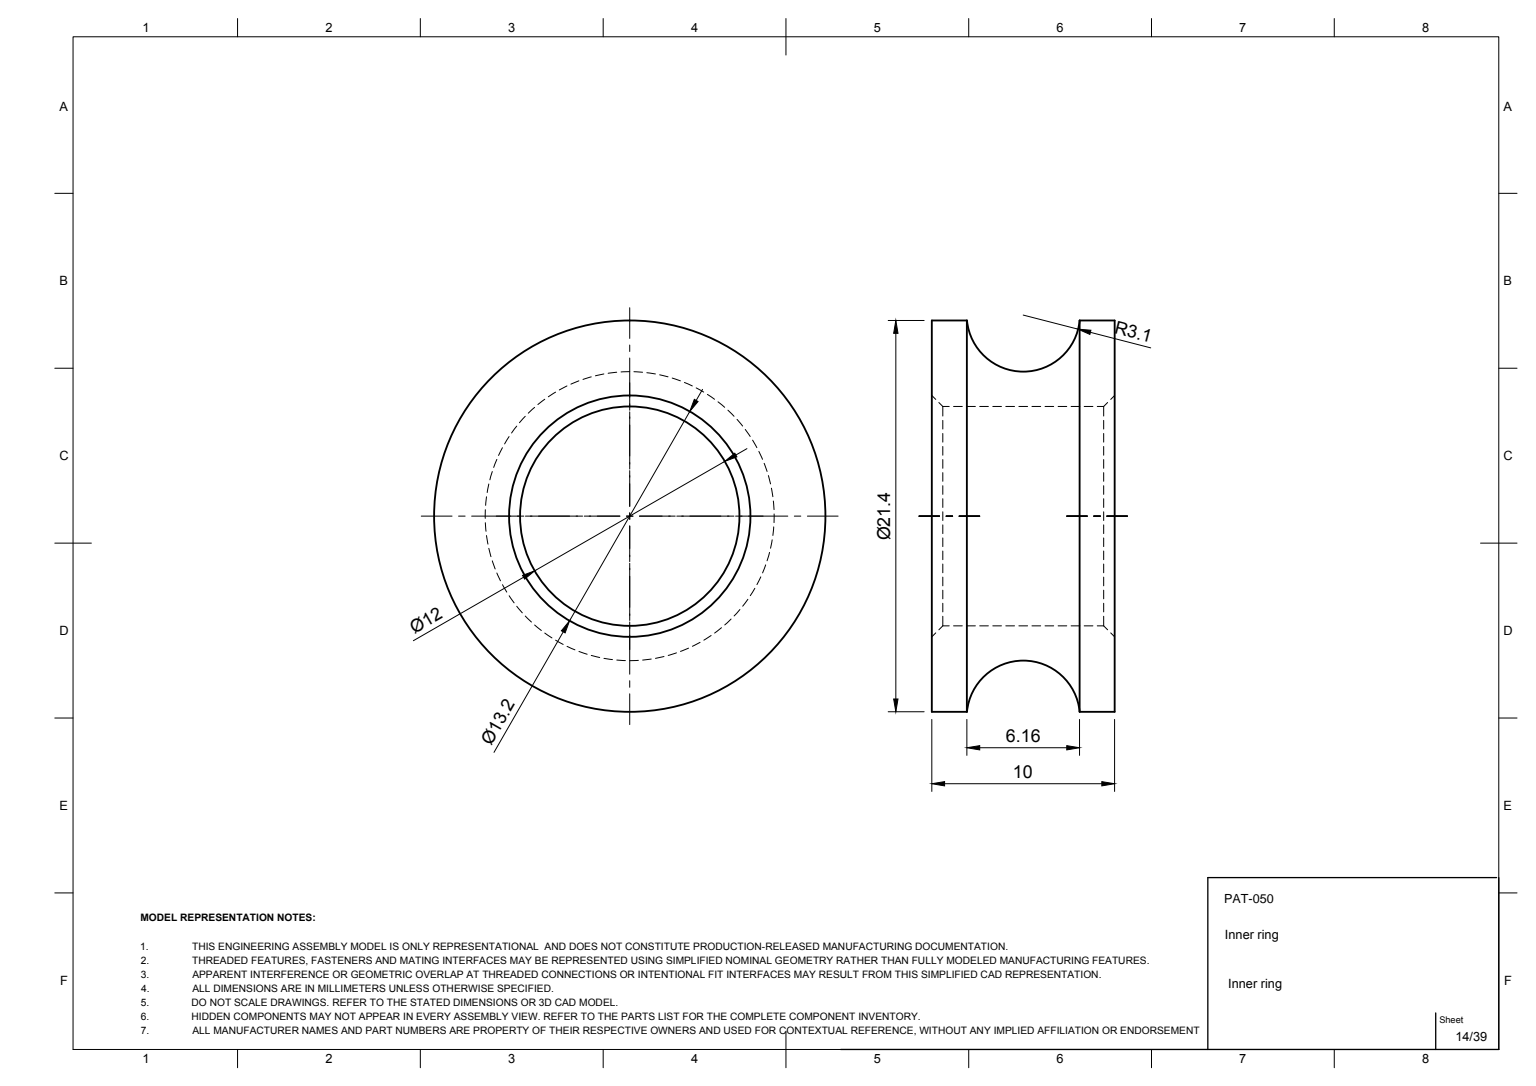
ISO-10303-21;
HEADER;
/* Generated by software containing ST-Developer
 * from STEP Tools, Inc. (www.steptools.com) 
 */

FILE_DESCRIPTION(
/* description */ ('Hand wheel with handle and shaft collar'),
/* implementation_level */ '2;1');

FILE_NAME(
/* name */ 'Inner ring.step',
/* time_stamp */ '2026-10-28T03:23:19-07:00',
/* author */ (''),
/* organization */ (''),
/* preprocessor_version */ 'ST-DEVELOPER v20.2',
/* originating_system */ 'Autodesk Translation Framework v15.17.0.0',
/* authorisation */ '');

FILE_SCHEMA (('AUTOMOTIVE_DESIGN { 1 0 10303 214 3 1 1 }'));
ENDSEC;

DATA;
#10=MECHANICAL_DESIGN_GEOMETRIC_PRESENTATION_REPRESENTATION('',(#404),#10510);
#297=TOROIDAL_SURFACE('',#5864,1.1,0.309556);
#304=CONICAL_SURFACE('',#5875,0.63,0.785398163397448);
#305=CONICAL_SURFACE('',#5882,0.63,0.785398163397448);
#340=SHAPE_REPRESENTATION_RELATIONSHIP('SRR','None',#10657,#372);
#372=ADVANCED_BREP_SHAPE_REPRESENTATION('',(#450),#10484);
#404=STYLED_ITEM('',(#10908),#450);
#450=MANIFOLD_SOLID_BREP('Body1',#5304);
#539=FACE_BOUND('',#1225,.T.);
#540=FACE_BOUND('',#1228,.T.);
#647=PLANE('',#5877);
#648=PLANE('',#5880);
#848=FACE_OUTER_BOUND('',#1220,.T.);
#849=FACE_OUTER_BOUND('',#1221,.T.);
#850=FACE_OUTER_BOUND('',#1222,.T.);
#851=FACE_OUTER_BOUND('',#1223,.T.);
#852=FACE_OUTER_BOUND('',#1224,.T.);
#853=FACE_OUTER_BOUND('',#1226,.T.);
#854=FACE_OUTER_BOUND('',#1227,.T.);
#855=FACE_OUTER_BOUND('',#1229,.T.);
#1220=EDGE_LOOP('',(#3923,#3924,#3925,#3926,#3927,#3928));
#1221=EDGE_LOOP('',(#3929,#3930,#3931,#3932,#3933));
#1222=EDGE_LOOP('',(#3934,#3935,#3936,#3937));
#1223=EDGE_LOOP('',(#3938,#3939,#3940,#3941));
#1224=EDGE_LOOP('',(#3942));
#1225=EDGE_LOOP('',(#3943));
#1226=EDGE_LOOP('',(#3944,#3945,#3946,#3947,#3948));
#1227=EDGE_LOOP('',(#3949));
#1228=EDGE_LOOP('',(#3950));
#1229=EDGE_LOOP('',(#3951,#3952,#3953,#3954));
#1627=LINE('',#8587,#1937);
#1628=LINE('',#8593,#1938);
#1629=LINE('',#8597,#1939);
#1630=LINE('',#8603,#1940);
#1631=LINE('',#8608,#1941);
#1937=VECTOR('',#6881,1.070235);
#1938=VECTOR('',#6888,0.6);
#1939=VECTOR('',#6893,0.63);
#1940=VECTOR('',#6902,1.070235);
#1941=VECTOR('',#6909,0.63);
#2202=CIRCLE('',#5865,1.070235);
#2203=CIRCLE('',#5866,1.070235);
#2204=CIRCLE('',#5867,0.309556);
#2205=CIRCLE('',#5868,1.070235);
#2206=CIRCLE('',#5869,1.070235);
#2207=CIRCLE('',#5871,1.070235);
#2208=CIRCLE('',#5873,0.6);
#2209=CIRCLE('',#5874,0.6);
#2210=CIRCLE('',#5876,0.66);
#2211=CIRCLE('',#5879,1.070235);
#2212=CIRCLE('',#5881,0.66);
#2565=VERTEX_POINT('',#8576);
#2566=VERTEX_POINT('',#8577);
#2567=VERTEX_POINT('',#8580);
#2568=VERTEX_POINT('',#8582);
#2569=VERTEX_POINT('',#8586);
#2570=VERTEX_POINT('',#8590);
#2571=VERTEX_POINT('',#8592);
#2572=VERTEX_POINT('',#8596);
#2573=VERTEX_POINT('',#8601);
#2574=VERTEX_POINT('',#8605);
#3079=EDGE_CURVE('',#2565,#2566,#2202,.T.);
#3080=EDGE_CURVE('',#2566,#2565,#2203,.T.);
#3081=EDGE_CURVE('',#2566,#2567,#2204,.T.);
#3082=EDGE_CURVE('',#2568,#2567,#2205,.T.);
#3083=EDGE_CURVE('',#2567,#2568,#2206,.T.);
#3084=EDGE_CURVE('',#2568,#2569,#1627,.T.);
#3085=EDGE_CURVE('',#2569,#2569,#2207,.T.);
#3086=EDGE_CURVE('',#2570,#2570,#2208,.T.);
#3087=EDGE_CURVE('',#2570,#2571,#1628,.T.);
#3088=EDGE_CURVE('',#2571,#2571,#2209,.T.);
#3089=EDGE_CURVE('',#2571,#2572,#1629,.T.);
#3090=EDGE_CURVE('',#2572,#2572,#2210,.T.);
#3091=EDGE_CURVE('',#2573,#2573,#2211,.T.);
#3092=EDGE_CURVE('',#2573,#2565,#1630,.T.);
#3093=EDGE_CURVE('',#2574,#2574,#2212,.T.);
#3094=EDGE_CURVE('',#2574,#2570,#1631,.T.);
#3923=ORIENTED_EDGE('',*,*,#3079,.F.);
#3924=ORIENTED_EDGE('',*,*,#3080,.F.);
#3925=ORIENTED_EDGE('',*,*,#3081,.T.);
#3926=ORIENTED_EDGE('',*,*,#3082,.F.);
#3927=ORIENTED_EDGE('',*,*,#3083,.F.);
#3928=ORIENTED_EDGE('',*,*,#3081,.F.);
#3929=ORIENTED_EDGE('',*,*,#3082,.T.);
#3930=ORIENTED_EDGE('',*,*,#3083,.T.);
#3931=ORIENTED_EDGE('',*,*,#3084,.T.);
#3932=ORIENTED_EDGE('',*,*,#3085,.T.);
#3933=ORIENTED_EDGE('',*,*,#3084,.F.);
#3934=ORIENTED_EDGE('',*,*,#3086,.T.);
#3935=ORIENTED_EDGE('',*,*,#3087,.T.);
#3936=ORIENTED_EDGE('',*,*,#3088,.F.);
#3937=ORIENTED_EDGE('',*,*,#3087,.F.);
#3938=ORIENTED_EDGE('',*,*,#3088,.T.);
#3939=ORIENTED_EDGE('',*,*,#3089,.T.);
#3940=ORIENTED_EDGE('',*,*,#3090,.F.);
#3941=ORIENTED_EDGE('',*,*,#3089,.F.);
#3942=ORIENTED_EDGE('',*,*,#3085,.F.);
#3943=ORIENTED_EDGE('',*,*,#3090,.T.);
#3944=ORIENTED_EDGE('',*,*,#3091,.F.);
#3945=ORIENTED_EDGE('',*,*,#3092,.T.);
#3946=ORIENTED_EDGE('',*,*,#3079,.T.);
#3947=ORIENTED_EDGE('',*,*,#3080,.T.);
#3948=ORIENTED_EDGE('',*,*,#3092,.F.);
#3949=ORIENTED_EDGE('',*,*,#3091,.T.);
#3950=ORIENTED_EDGE('',*,*,#3093,.F.);
#3951=ORIENTED_EDGE('',*,*,#3093,.T.);
#3952=ORIENTED_EDGE('',*,*,#3094,.T.);
#3953=ORIENTED_EDGE('',*,*,#3086,.F.);
#3954=ORIENTED_EDGE('',*,*,#3094,.F.);
#4912=CYLINDRICAL_SURFACE('',#5870,1.070235);
#4913=CYLINDRICAL_SURFACE('',#5872,0.6);
#4914=CYLINDRICAL_SURFACE('',#5878,1.070235);
#5060=ADVANCED_FACE('',(#848),#297,.F.);
#5061=ADVANCED_FACE('',(#849),#4912,.T.);
#5062=ADVANCED_FACE('',(#850),#4913,.F.);
#5063=ADVANCED_FACE('',(#851),#304,.F.);
#5064=ADVANCED_FACE('',(#852,#539),#647,.T.);
#5065=ADVANCED_FACE('',(#853),#4914,.T.);
#5066=ADVANCED_FACE('',(#854,#540),#648,.T.);
#5067=ADVANCED_FACE('',(#855),#305,.F.);
#5304=CLOSED_SHELL('',(#5060,#5061,#5062,#5063,#5064,#5065,#5066,#5067));
#5863=AXIS2_PLACEMENT_3D('',#8574,#6865,#6866);
#5864=AXIS2_PLACEMENT_3D('',#8575,#6867,#6868);
#5865=AXIS2_PLACEMENT_3D('',#8578,#6869,#6870);
#5866=AXIS2_PLACEMENT_3D('',#8579,#6871,#6872);
#5867=AXIS2_PLACEMENT_3D('',#8581,#6873,#6874);
#5868=AXIS2_PLACEMENT_3D('',#8583,#6875,#6876);
#5869=AXIS2_PLACEMENT_3D('',#8584,#6877,#6878);
#5870=AXIS2_PLACEMENT_3D('',#8585,#6879,#6880);
#5871=AXIS2_PLACEMENT_3D('',#8588,#6882,#6883);
#5872=AXIS2_PLACEMENT_3D('',#8589,#6884,#6885);
#5873=AXIS2_PLACEMENT_3D('',#8591,#6886,#6887);
#5874=AXIS2_PLACEMENT_3D('',#8594,#6889,#6890);
#5875=AXIS2_PLACEMENT_3D('',#8595,#6891,#6892);
#5876=AXIS2_PLACEMENT_3D('',#8598,#6894,#6895);
#5877=AXIS2_PLACEMENT_3D('',#8599,#6896,#6897);
#5878=AXIS2_PLACEMENT_3D('',#8600,#6898,#6899);
#5879=AXIS2_PLACEMENT_3D('',#8602,#6900,#6901);
#5880=AXIS2_PLACEMENT_3D('',#8604,#6903,#6904);
#5881=AXIS2_PLACEMENT_3D('',#8606,#6905,#6906);
#5882=AXIS2_PLACEMENT_3D('',#8607,#6907,#6908);
#6865=DIRECTION('axis',(0.,0.,1.));
#6866=DIRECTION('refdir',(1.,0.,0.));
#6867=DIRECTION('center_axis',(0.,-1.,0.));
#6868=DIRECTION('ref_axis',(0.,0.,-1.));
#6869=DIRECTION('center_axis',(0.,-1.,0.));
#6870=DIRECTION('ref_axis',(1.,0.,0.));
#6871=DIRECTION('center_axis',(0.,-1.,0.));
#6872=DIRECTION('ref_axis',(1.,0.,0.));
#6873=DIRECTION('center_axis',(1.,0.,1.22464679914735E-16));
#6874=DIRECTION('ref_axis',(-1.22464679914735E-16,0.,1.));
#6875=DIRECTION('center_axis',(0.,1.,0.));
#6876=DIRECTION('ref_axis',(1.,0.,0.));
#6877=DIRECTION('center_axis',(0.,1.,0.));
#6878=DIRECTION('ref_axis',(1.,0.,0.));
#6879=DIRECTION('center_axis',(0.,-1.,0.));
#6880=DIRECTION('ref_axis',(1.,0.,0.));
#6881=DIRECTION('',(0.,1.,0.));
#6882=DIRECTION('center_axis',(0.,-1.,0.));
#6883=DIRECTION('ref_axis',(1.,0.,0.));
#6884=DIRECTION('center_axis',(0.,-1.,0.));
#6885=DIRECTION('ref_axis',(1.,0.,0.));
#6886=DIRECTION('center_axis',(0.,-1.,0.));
#6887=DIRECTION('ref_axis',(1.,0.,0.));
#6888=DIRECTION('',(0.,1.,0.));
#6889=DIRECTION('center_axis',(0.,-1.,0.));
#6890=DIRECTION('ref_axis',(1.,0.,0.));
#6891=DIRECTION('center_axis',(0.,1.,0.));
#6892=DIRECTION('ref_axis',(1.,0.,0.));
#6893=DIRECTION('',(-0.707106781186548,0.707106781186547,-8.65956056235493E-17));
#6894=DIRECTION('center_axis',(0.,-1.,0.));
#6895=DIRECTION('ref_axis',(1.,0.,0.));
#6896=DIRECTION('center_axis',(0.,1.,0.));
#6897=DIRECTION('ref_axis',(0.,0.,1.));
#6898=DIRECTION('center_axis',(0.,-1.,0.));
#6899=DIRECTION('ref_axis',(1.,0.,0.));
#6900=DIRECTION('center_axis',(0.,-1.,0.));
#6901=DIRECTION('ref_axis',(1.,0.,0.));
#6902=DIRECTION('',(0.,1.,0.));
#6903=DIRECTION('center_axis',(0.,-1.,0.));
#6904=DIRECTION('ref_axis',(0.,0.,-1.));
#6905=DIRECTION('center_axis',(0.,-1.,0.));
#6906=DIRECTION('ref_axis',(1.,0.,0.));
#6907=DIRECTION('center_axis',(0.,-1.,0.));
#6908=DIRECTION('ref_axis',(1.,0.,0.));
#6909=DIRECTION('',(0.707106781186548,0.707106781186547,8.65956056235493E-17));
#8574=CARTESIAN_POINT('',(0.,0.,0.));
#8575=CARTESIAN_POINT('Origin',(0.,0.,0.));
#8576=CARTESIAN_POINT('',(-1.070235,-0.308121667383195,-1.31065986708547E-16));
#8577=CARTESIAN_POINT('',(-1.31065986708547E-16,-0.308121667383195,1.070235));
#8578=CARTESIAN_POINT('Origin',(0.,-0.308121667383195,0.));
#8579=CARTESIAN_POINT('Origin',(0.,-0.308121667383195,0.));
#8580=CARTESIAN_POINT('',(-1.31065986708547E-16,0.308121667383195,1.070235));
#8581=CARTESIAN_POINT('Origin',(-1.34711147906209E-16,0.,1.1));
#8582=CARTESIAN_POINT('',(-1.070235,0.308121667383195,1.31065986708547E-16));
#8583=CARTESIAN_POINT('Origin',(0.,0.308121667383195,0.));
#8584=CARTESIAN_POINT('Origin',(0.,0.308121667383195,0.));
#8585=CARTESIAN_POINT('Origin',(0.,0.,0.));
#8586=CARTESIAN_POINT('',(-1.070235,0.5,-1.31065986708547E-16));
#8587=CARTESIAN_POINT('',(-1.070235,0.,-1.31065986708547E-16));
#8588=CARTESIAN_POINT('Origin',(0.,0.5,0.));
#8589=CARTESIAN_POINT('Origin',(0.,0.,0.));
#8590=CARTESIAN_POINT('',(-0.6,-0.44,-7.34788079488412E-17));
#8591=CARTESIAN_POINT('Origin',(0.,-0.44,0.));
#8592=CARTESIAN_POINT('',(-0.6,0.44,-7.34788079488412E-17));
#8593=CARTESIAN_POINT('',(-0.6,0.,-7.34788079488412E-17));
#8594=CARTESIAN_POINT('Origin',(0.,0.44,0.));
#8595=CARTESIAN_POINT('Origin',(0.,0.47,0.));
#8596=CARTESIAN_POINT('',(-0.66,0.5,-8.08266887437253E-17));
#8597=CARTESIAN_POINT('',(-0.63,0.47,-7.71527483462832E-17));
#8598=CARTESIAN_POINT('Origin',(0.,0.5,0.));
#8599=CARTESIAN_POINT('Origin',(1.070235,0.5,0.));
#8600=CARTESIAN_POINT('Origin',(0.,0.,0.));
#8601=CARTESIAN_POINT('',(-1.070235,-0.5,-1.31065986708547E-16));
#8602=CARTESIAN_POINT('Origin',(0.,-0.5,0.));
#8603=CARTESIAN_POINT('',(-1.070235,0.,-1.31065986708547E-16));
#8604=CARTESIAN_POINT('Origin',(0.66,-0.5,0.));
#8605=CARTESIAN_POINT('',(-0.66,-0.5,-8.08266887437253E-17));
#8606=CARTESIAN_POINT('Origin',(0.,-0.5,0.));
#8607=CARTESIAN_POINT('Origin',(0.,-0.47,0.));
#8608=CARTESIAN_POINT('',(-0.63,-0.47,-7.71527483462832E-17));
#10445=UNCERTAINTY_MEASURE_WITH_UNIT(LENGTH_MEASURE(0.001),#10511,
'DISTANCE_ACCURACY_VALUE',
'Maximum model space distance between geometric entities at asserted c
onnectivities');
#10471=UNCERTAINTY_MEASURE_WITH_UNIT(LENGTH_MEASURE(0.001),#10511,
'DISTANCE_ACCURACY_VALUE',
'Maximum model space distance between geometric entities at asserted c
onnectivities');
#10484=(
GEOMETRIC_REPRESENTATION_CONTEXT(3)
GLOBAL_UNCERTAINTY_ASSIGNED_CONTEXT((#10445))
GLOBAL_UNIT_ASSIGNED_CONTEXT((#10511,#10513,#10514))
REPRESENTATION_CONTEXT('','3D')
);
#10510=(
GEOMETRIC_REPRESENTATION_CONTEXT(3)
GLOBAL_UNCERTAINTY_ASSIGNED_CONTEXT((#10471))
GLOBAL_UNIT_ASSIGNED_CONTEXT((#10511,#10513,#10514))
REPRESENTATION_CONTEXT('','3D')
);
#10511=(
LENGTH_UNIT()
NAMED_UNIT(*)
SI_UNIT(.CENTI.,.METRE.)
);
#10513=(
NAMED_UNIT(*)
PLANE_ANGLE_UNIT()
SI_UNIT($,.RADIAN.)
);
#10514=(
NAMED_UNIT(*)
SI_UNIT($,.STERADIAN.)
SOLID_ANGLE_UNIT()
);
#10527=SHAPE_DEFINITION_REPRESENTATION(#10565,#10657);
#10565=PRODUCT_DEFINITION_SHAPE('',$,#10696);
#10657=SHAPE_REPRESENTATION('',(#5863),#10484);
#10683=PRODUCT_DEFINITION_CONTEXT('part definition',#10799,'design');
#10696=PRODUCT_DEFINITION('Inner ring','Inner ring',#10734,#10683);
#10734=PRODUCT_DEFINITION_FORMATION('',$,#10813);
#10799=APPLICATION_CONTEXT(
'Core Data for Automotive Mechanical Design Process');
#10800=PRODUCT_CONTEXT('part definition',#10799,'mechanical');
#10813=PRODUCT('Inner ring','Inner ring','Inner ring',(#10800));
#10902=COLOUR_RGB('Grey',0.48,0.52,0.57);
#10903=FILL_AREA_STYLE_COLOUR('',#10902);
#10904=FILL_AREA_STYLE('',(#10903));
#10905=SURFACE_STYLE_FILL_AREA(#10904);
#10906=SURFACE_SIDE_STYLE('',(#10905));
#10907=SURFACE_STYLE_USAGE(.BOTH.,#10906);
#10908=PRESENTATION_STYLE_ASSIGNMENT((#10907));
ENDSEC;
END-ISO-10303-21;
